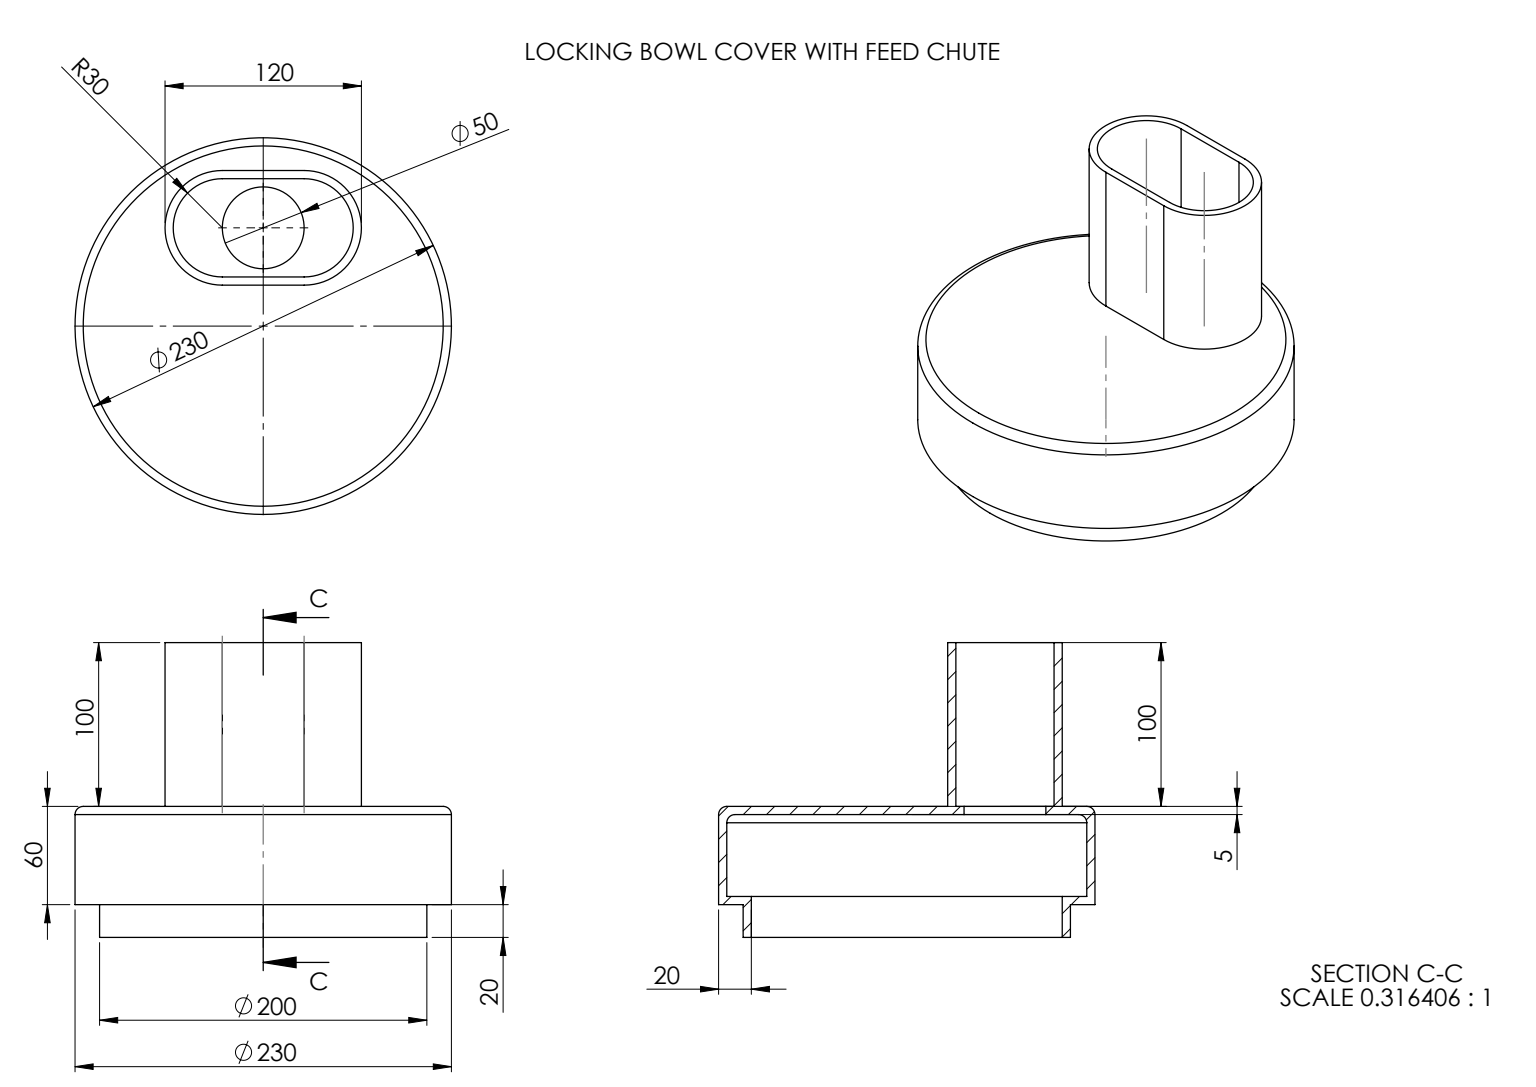
ISO-10303-21;
HEADER;
FILE_DESCRIPTION (('STEP AP214'),
    '1' );
FILE_NAME ('Locking Bowl Cover with Feed Chute.step',
    '2026-10-08T14:59:03',
    ( '' ),
    ( '' ),
    'SwSTEP 2.0',
    'SolidWorks 2026',
    '' );
FILE_SCHEMA (( 'AUTOMOTIVE_DESIGN' ));
ENDSEC;

DATA;
#12=CARTESIAN_POINT ( 'NONE',  ( -25.00000000000000000, 445.0000000000000568, -90.00000000000000000 ) ) ;
#55=DIRECTION ( 'NONE',  ( -0.000000000000000000, -1.000000000000000000, -0.000000000000000000 ) ) ;
#62=CARTESIAN_POINT ( 'NONE',  ( -25.00000000000000000, 345.0000000000000568, -90.00000000000000000 ) ) ;
#72=FACE_BOUND ( 'NONE', #11694, .T. ) ;
#91=EDGE_CURVE ( 'NONE', #9396, #343, #11975, .T. ) ;
#93=VECTOR ( 'NONE', #163, 1000.000000000000000 ) ;
#95=AXIS2_PLACEMENT_3D ( 'NONE', #7431, #12111, #3682 ) ;
#112=AXIS2_PLACEMENT_3D ( 'NONE', #12229, #2739, #12169 ) ;
#129=ORIENTED_EDGE ( 'NONE', *, *, #8171, .F. ) ;
#161=CARTESIAN_POINT ( 'NONE',  ( 0.000000000000000000, 264.9990000000000236, -34.99999999999999289 ) ) ;
#163=DIRECTION ( 'NONE',  ( -0.000000000000000000, -1.000000000000000000, -0.000000000000000000 ) ) ;
#170=ORIENTED_EDGE ( 'NONE', *, *, #8169, .T. ) ;
#173=EDGE_LOOP ( 'NONE', ( #129, #2028 ) ) ;
#209=EDGE_LOOP ( 'NONE', ( #9146, #6174, #8156, #10356 ) ) ;
#241=EDGE_LOOP ( 'NONE', ( #9519, #6626 ) ) ;
#258=ORIENTED_EDGE ( 'NONE', *, *, #4138, .F. ) ;
#290=ORIENTED_EDGE ( 'NONE', *, *, #11197, .T. ) ;
#300=DIRECTION ( 'NONE',  ( 0.000000000000000000, 1.000000000000000000, 0.000000000000000000 ) ) ;
#319=CARTESIAN_POINT ( 'NONE',  ( 25.00000000000000000, 445.0000000000000568, -59.99999999999999289 ) ) ;
#338=EDGE_CURVE ( 'NONE', #9423, #8980, #11374, .T. ) ;
#343=VERTEX_POINT ( 'NONE', #2827 ) ;
#362=ORIENTED_EDGE ( 'NONE', *, *, #8065, .F. ) ;
#365=EDGE_CURVE ( 'NONE', #6665, #9990, #8676, .T. ) ;
#366=VERTEX_POINT ( 'NONE', #3827 ) ;
#395=CARTESIAN_POINT ( 'NONE',  ( 0.000000000000000000, 290.0000000000000568, 0.000000000000000000 ) ) ;
#414=CARTESIAN_POINT ( 'NONE',  ( -25.00000000000000000, 445.0000000000000568, -24.99999999999998934 ) ) ;
#450=ORIENTED_EDGE ( 'NONE', *, *, #10797, .T. ) ;
#463=( LENGTH_UNIT ( ) NAMED_UNIT ( * ) SI_UNIT ( .MILLI., .METRE. ) );
#483=VECTOR ( 'NONE', #12060, 1000.000000000000000 ) ;
#559=EDGE_CURVE ( 'NONE', #12107, #9423, #10128, .T. ) ;
#569=FACE_OUTER_BOUND ( 'NONE', #2899, .T. ) ;
#606=AXIS2_PLACEMENT_3D ( 'NONE', #1785, #8264, #12267 ) ;
#623=CIRCLE ( 'NONE', #4397, 100.0000000000000284 ) ;
#634=CARTESIAN_POINT ( 'NONE',  ( 0.000000000000000000, 340.0000000000000000, 0.000000000000000000 ) ) ;
#645=DIRECTION ( 'NONE',  ( 0.000000000000000000, -0.000000000000000000, 1.000000000000000000 ) ) ;
#656=ORIENTED_EDGE ( 'NONE', *, *, #8171, .T. ) ;
#660=CARTESIAN_POINT ( 'NONE',  ( 0.000000000000000000, 264.9990000000000236, -59.99999999999999289 ) ) ;
#673=ORIENTED_EDGE ( 'NONE', *, *, #10831, .F. ) ;
#749=EDGE_CURVE ( 'NONE', #980, #10107, #8125, .T. ) ;
#766=LINE ( 'NONE', #6554, #1224 ) ;
#768=EDGE_LOOP ( 'NONE', ( #10087, #10275, #11943, #656 ) ) ;
#775=EDGE_CURVE ( 'NONE', #8980, #6431, #10558, .T. ) ;
#792=CARTESIAN_POINT ( 'NONE',  ( 24.99999999999999645, 445.0000000000000568, -95.00000000000000000 ) ) ;
#795=CARTESIAN_POINT ( 'NONE',  ( -25.00000000000000000, 445.0000000000000568, -90.00000000000000000 ) ) ;
#797=DIRECTION ( 'NONE',  ( -0.000000000000000000, -1.000000000000000000, -0.000000000000000000 ) ) ;
#798=ADVANCED_FACE ( 'NONE', ( #9554 ), #9306, .F. ) ;
#799=AXIS2_PLACEMENT_3D ( 'NONE', #8396, #2668, #933 ) ;
#809=CARTESIAN_POINT ( 'NONE',  ( 0.000000000000000000, 265.0000000000000000, 0.000000000000000000 ) ) ;
#826=AXIS2_PLACEMENT_3D ( 'NONE', #4284, #9299, #12253 ) ;
#839=ORIENTED_EDGE ( 'NONE', *, *, #3131, .F. ) ;
#842=VECTOR ( 'NONE', #3095, 1000.000000000000000 ) ;
#857=DIRECTION ( 'NONE',  ( 0.000000000000000000, 0.000000000000000000, -1.000000000000000000 ) ) ;
#868=VECTOR ( 'NONE', #6176, 1000.000000000000000 ) ;
#878=ORIENTED_EDGE ( 'NONE', *, *, #1877, .T. ) ;
#910=CARTESIAN_POINT ( 'NONE',  ( -25.00000000000000000, 445.0000000000000568, -90.00000000000000000 ) ) ;
#920=DIRECTION ( 'NONE',  ( -0.000000000000000000, -1.000000000000000000, -0.000000000000000000 ) ) ;
#932=DIRECTION ( 'NONE',  ( 0.000000000000000000, 0.000000000000000000, 1.000000000000000000 ) ) ;
#933=DIRECTION ( 'NONE',  ( 0.000000000000000000, 0.000000000000000000, 1.000000000000000000 ) ) ;
#962=DIRECTION ( 'NONE',  ( 0.000000000000000000, 1.000000000000000000, 0.000000000000000000 ) ) ;
#971=ORIENTED_EDGE ( 'NONE', *, *, #3981, .F. ) ;
#980=VERTEX_POINT ( 'NONE', #1154 ) ;
#994=MECHANICAL_DESIGN_GEOMETRIC_PRESENTATION_REPRESENTATION('',(#6364),#3151);
#1004=VERTEX_POINT ( 'NONE', #10865 ) ;
#1020=DIRECTION ( 'NONE',  ( -0.000000000000000000, -1.000000000000000000, -0.000000000000000000 ) ) ;
#1022=EDGE_CURVE ( 'NONE', #1669, #6843, #3206, .T. ) ;
#1047=ORIENTED_EDGE ( 'NONE', *, *, #3864, .F. ) ;
#1059=CARTESIAN_POINT ( 'NONE',  ( 0.000000000000000000, 335.0000000000000000, 0.000000000000000000 ) ) ;
#1066=CARTESIAN_POINT ( 'NONE',  ( 0.000000000000000000, 340.0000000000000000, 0.000000000000000000 ) ) ;
#1080=EDGE_CURVE ( 'NONE', #366, #8042, #4441, .T. ) ;
#1100=CIRCLE ( 'NONE', #7062, 25.00000000000000000 ) ;
#1103=ORIENTED_EDGE ( 'NONE', *, *, #4649, .T. ) ;
#1110=CARTESIAN_POINT ( 'NONE',  ( -25.00000000000000000, 445.0000000000000568, -29.99999999999999289 ) ) ;
#1114=PRODUCT_DEFINITION_SHAPE ( 'NONE', 'NONE',  #7780 ) ;
#1116=AXIS2_PLACEMENT_3D ( 'NONE', #2438, #7051, #1380 ) ;
#1128=ORIENTED_EDGE ( 'NONE', *, *, #4703, .F. ) ;
#1129=DIRECTION ( 'NONE',  ( 0.000000000000000000, 0.000000000000000000, 1.000000000000000000 ) ) ;
#1131=CARTESIAN_POINT ( 'NONE',  ( 0.000000000000000000, 340.0000000000000000, 0.000000000000000000 ) ) ;
#1154=CARTESIAN_POINT ( 'NONE',  ( 3.061616997868383043E-15, 340.0000000000000000, -84.99999999999998579 ) ) ;
#1180=DIRECTION ( 'NONE',  ( 0.000000000000000000, 0.000000000000000000, -1.000000000000000000 ) ) ;
#1192=CARTESIAN_POINT ( 'NONE',  ( 0.000000000000000000, 265.0000000000000000, 0.000000000000000000 ) ) ;
#1193=ORIENTED_EDGE ( 'NONE', *, *, #4561, .T. ) ;
#1196=ORIENTED_EDGE ( 'NONE', *, *, #3655, .T. ) ;
#1224=VECTOR ( 'NONE', #12235, 1000.000000000000000 ) ;
#1227=DIRECTION ( 'NONE',  ( 0.000000000000000000, 0.000000000000000000, 1.000000000000000000 ) ) ;
#1238=AXIS2_PLACEMENT_3D ( 'NONE', #1784, #6529, #6582 ) ;
#1248=AXIS2_PLACEMENT_3D ( 'NONE', #10310, #6332, #2532 ) ;
#1250=DIRECTION ( 'NONE',  ( 0.000000000000000000, 1.000000000000000000, 0.000000000000000000 ) ) ;
#1292=DIRECTION ( 'NONE',  ( 1.000000000000000000, 0.000000000000000000, -0.000000000000000000 ) ) ;
#1297=LINE ( 'NONE', #10769, #9355 ) ;
#1313=CLOSED_SHELL ( 'NONE', ( #3230, #7953, #9387, #12328, #9620, #5138, #7591, #4251, #2390, #5665, #9897, #798, #10427, #12260, #12222, #2538, #10180, #10873, #5121, #9944, #12231, #11960, #6025, #4909, #4674, #5505, #5178, #3185, #9915 ) ) ;
#1315=CIRCLE ( 'NONE', #5902, 35.00000000000000000 ) ;
#1317=ORIENTED_EDGE ( 'NONE', *, *, #9120, .T. ) ;
#1325=CYLINDRICAL_SURFACE ( 'NONE', #1672, 95.00000000000002842 ) ;
#1346=ORIENTED_EDGE ( 'NONE', *, *, #5064, .F. ) ;
#1380=DIRECTION ( 'NONE',  ( 0.000000000000000000, 0.000000000000000000, 1.000000000000000000 ) ) ;
#1381=ORIENTED_EDGE ( 'NONE', *, *, #10829, .T. ) ;
#1410=CARTESIAN_POINT ( 'NONE',  ( 0.000000000000000000, 340.0000000000000000, 0.000000000000000000 ) ) ;
#1422=VECTOR ( 'NONE', #9629, 1000.000000000000000 ) ;
#1427=DIRECTION ( 'NONE',  ( 0.000000000000000000, 1.000000000000000000, 0.000000000000000000 ) ) ;
#1464=PLANE ( 'NONE',  #3000 ) ;
#1475=DIRECTION ( 'NONE',  ( -0.000000000000000000, -1.000000000000000000, -0.000000000000000000 ) ) ;
#1478=DIRECTION ( 'NONE',  ( 0.000000000000000000, 0.000000000000000000, 1.000000000000000000 ) ) ;
#1485=EDGE_LOOP ( 'NONE', ( #5479, #1619 ) ) ;
#1488=CARTESIAN_POINT ( 'NONE',  ( 0.000000000000000000, 345.0000000000000568, -59.99999999999999289 ) ) ;
#1495=ORIENTED_EDGE ( 'NONE', *, *, #3254, .F. ) ;
#1496=DIRECTION ( 'NONE',  ( 0.000000000000000000, 0.000000000000000000, 1.000000000000000000 ) ) ;
#1516=EDGE_CURVE ( 'NONE', #9990, #4918, #10969, .T. ) ;
#1579=DIRECTION ( 'NONE',  ( 0.000000000000000000, 0.000000000000000000, 1.000000000000000000 ) ) ;
#1584=DIRECTION ( 'NONE',  ( 0.000000000000000000, 0.000000000000000000, 1.000000000000000000 ) ) ;
#1588=EDGE_CURVE ( 'NONE', #6133, #7105, #5611, .T. ) ;
#1591=SURFACE_STYLE_USAGE ( .BOTH. , #4385 ) ;
#1592=CIRCLE ( 'NONE', #2182, 110.0000000000000284 ) ;
#1594=FACE_OUTER_BOUND ( 'NONE', #6328, .T. ) ;
#1610=AXIS2_PLACEMENT_3D ( 'NONE', #11271, #10315, #5592 ) ;
#1612=AXIS2_PLACEMENT_3D ( 'NONE', #9562, #7823, #5032 ) ;
#1618=DIRECTION ( 'NONE',  ( 0.000000000000000000, 0.000000000000000000, 1.000000000000000000 ) ) ;
#1619=ORIENTED_EDGE ( 'NONE', *, *, #3254, .T. ) ;
#1647=ORIENTED_EDGE ( 'NONE', *, *, #9120, .F. ) ;
#1648=CARTESIAN_POINT ( 'NONE',  ( 25.00000000000000000, 345.0000000000000568, -24.99999999999998934 ) ) ;
#1668=DIRECTION ( 'NONE',  ( 0.000000000000000000, 0.000000000000000000, -1.000000000000000000 ) ) ;
#1669=VERTEX_POINT ( 'NONE', #3557 ) ;
#1672=AXIS2_PLACEMENT_3D ( 'NONE', #10853, #2316, #5437 ) ;
#1683=AXIS2_PLACEMENT_3D ( 'NONE', #10392, #1855, #932 ) ;
#1687=ORIENTED_EDGE ( 'NONE', *, *, #11584, .F. ) ;
#1702=VECTOR ( 'NONE', #8940, 1000.000000000000000 ) ;
#1713=DIRECTION ( 'NONE',  ( 0.000000000000000000, -0.000000000000000000, 1.000000000000000000 ) ) ;
#1751=EDGE_CURVE ( 'NONE', #2693, #6100, #5845, .T. ) ;
#1784=CARTESIAN_POINT ( 'NONE',  ( 0.000000000000000000, 264.9990000000000236, -59.99999999999999289 ) ) ;
#1785=CARTESIAN_POINT ( 'NONE',  ( -25.00000000000000000, 445.0000000000000568, -59.99999999999999289 ) ) ;
#1844=CARTESIAN_POINT ( 'NONE',  ( 0.000000000000000000, 340.0000000000000000, 0.000000000000000000 ) ) ;
#1850=DIRECTION ( 'NONE',  ( -1.000000000000000000, 0.000000000000000000, 0.000000000000000000 ) ) ;
#1855=DIRECTION ( 'NONE',  ( -0.000000000000000000, -1.000000000000000000, -0.000000000000000000 ) ) ;
#1859=CARTESIAN_POINT ( 'NONE',  ( -25.00000000000000000, 445.0000000000000568, -59.99999999999999289 ) ) ;
#1862=LINE ( 'NONE', #8522, #4334 ) ;
#1866=DIRECTION ( 'NONE',  ( 1.000000000000000000, 0.000000000000000000, 0.000000000000000000 ) ) ;
#1877=EDGE_CURVE ( 'NONE', #11984, #12107, #2341, .T. ) ;
#1899=PRODUCT ( 'Locking Bowl Cover with Feed Chute', 'Locking Bowl Cover with Feed Chute', '', ( #8716 ) ) ;
#1911=AXIS2_PLACEMENT_3D ( 'NONE', #10684, #11693, #3144 ) ;
#1940=DIRECTION ( 'NONE',  ( 1.000000000000000000, 0.000000000000000000, 0.000000000000000000 ) ) ;
#1958=EDGE_CURVE ( 'NONE', #12281, #3955, #5339, .T. ) ;
#1961=DIRECTION ( 'NONE',  ( -0.000000000000000000, -1.000000000000000000, -0.000000000000000000 ) ) ;
#1977=DIRECTION ( 'NONE',  ( 0.000000000000000000, 0.000000000000000000, 1.000000000000000000 ) ) ;
#1986=CARTESIAN_POINT ( 'NONE',  ( -25.00000000000000000, 445.0000000000000568, -29.99999999999999289 ) ) ;
#2004=AXIS2_PLACEMENT_3D ( 'NONE', #8641, #10522, #1180 ) ;
#2024=TOROIDAL_SURFACE ( 'NONE', #8969, 110.0000000000000284, 5.000000000000000000 ) ;
#2028=ORIENTED_EDGE ( 'NONE', *, *, #7862, .F. ) ;
#2060=DIRECTION ( 'NONE',  ( 0.000000000000000000, 1.000000000000000000, 0.000000000000000000 ) ) ;
#2064=VERTEX_POINT ( 'NONE', #9558 ) ;
#2098=AXIS2_PLACEMENT_3D ( 'NONE', #2517, #5324, #1579 ) ;
#2117=FACE_OUTER_BOUND ( 'NONE', #209, .T. ) ;
#2138=CARTESIAN_POINT ( 'NONE',  ( 1.408343819019456413E-14, 285.0000000000000568, 115.0000000000000284 ) ) ;
#2142=LINE ( 'NONE', #2197, #2388 ) ;
#2182=AXIS2_PLACEMENT_3D ( 'NONE', #2553, #6356, #1496 ) ;
#2197=CARTESIAN_POINT ( 'NONE',  ( -25.00000000000000000, 445.0000000000000568, -24.99999999999998934 ) ) ;
#2213=AXIS2_PLACEMENT_3D ( 'NONE', #1131, #55, #10532 ) ;
#2262=AXIS2_PLACEMENT_3D ( 'NONE', #3647, #12199, #5711 ) ;
#2263=AXIS2_PLACEMENT_3D ( 'NONE', #6307, #4185, #3445 ) ;
#2269=DIRECTION ( 'NONE',  ( 0.000000000000000000, 0.000000000000000000, 1.000000000000000000 ) ) ;
#2285=( LENGTH_UNIT ( ) NAMED_UNIT ( * ) SI_UNIT ( .MILLI., .METRE. ) );
#2301=CARTESIAN_POINT ( 'NONE',  ( -25.00000000000000000, 445.0000000000000568, -59.99999999999999289 ) ) ;
#2316=DIRECTION ( 'NONE',  ( 0.000000000000000000, 1.000000000000000000, 0.000000000000000000 ) ) ;
#2341=LINE ( 'NONE', #4034, #842 ) ;
#2342=PRESENTATION_STYLE_ASSIGNMENT (( #11772 ) ) ;
#2355=DIRECTION ( 'NONE',  ( 0.000000000000000000, 1.000000000000000000, 0.000000000000000000 ) ) ;
#2365=ORIENTED_EDGE ( 'NONE', *, *, #1877, .F. ) ;
#2388=VECTOR ( 'NONE', #5945, 1000.000000000000000 ) ;
#2389=FACE_OUTER_BOUND ( 'NONE', #3479, .T. ) ;
#2390=ADVANCED_FACE ( 'NONE', ( #10930, #2389 ), #1464, .T. ) ;
#2394=ORIENTED_EDGE ( 'NONE', *, *, #8117, .F. ) ;
#2438=CARTESIAN_POINT ( 'NONE',  ( 0.000000000000000000, 335.0000000000000000, 105.0000000000000284 ) ) ;
#2462=( NAMED_UNIT ( * ) PLANE_ANGLE_UNIT ( ) SI_UNIT ( $, .RADIAN. ) );
#2476=DIRECTION ( 'NONE',  ( 1.000000000000000000, 0.000000000000000000, 0.000000000000000000 ) ) ;
#2484=ORIENTED_EDGE ( 'NONE', *, *, #1751, .T. ) ;
#2514=CIRCLE ( 'NONE', #6297, 95.00000000000002842 ) ;
#2516=FACE_BOUND ( 'NONE', #241, .T. ) ;
#2517=CARTESIAN_POINT ( 'NONE',  ( 0.000000000000000000, 340.0000000000000000, -59.99999999999999289 ) ) ;
#2532=DIRECTION ( 'NONE',  ( 0.000000000000000000, 0.000000000000000000, 1.000000000000000000 ) ) ;
#2538=ADVANCED_FACE ( 'NONE', ( #2516, #12121 ), #5633, .F. ) ;
#2553=CARTESIAN_POINT ( 'NONE',  ( 0.000000000000000000, 335.0000000000000000, 0.000000000000000000 ) ) ;
#2595=EDGE_CURVE ( 'NONE', #10953, #6431, #2877, .T. ) ;
#2601=DIRECTION ( 'NONE',  ( -0.000000000000000000, -1.000000000000000000, -0.000000000000000000 ) ) ;
#2607=VERTEX_POINT ( 'NONE', #11365 ) ;
#2635=EDGE_LOOP ( 'NONE', ( #7285, #5878, #878, #11411 ) ) ;
#2643=EDGE_LOOP ( 'NONE', ( #5773, #6443, #6520, #10027 ) ) ;
#2668=DIRECTION ( 'NONE',  ( -0.000000000000000000, -1.000000000000000000, -0.000000000000000000 ) ) ;
#2681=AXIS2_PLACEMENT_3D ( 'NONE', #11662, #3113, #7033 ) ;
#2693=VERTEX_POINT ( 'NONE', #11425 ) ;
#2696=ORIENTED_EDGE ( 'NONE', *, *, #7107, .F. ) ;
#2718=CYLINDRICAL_SURFACE ( 'NONE', #8556, 110.0000000000000284 ) ;
#2739=DIRECTION ( 'NONE',  ( 0.000000000000000000, 1.000000000000000000, 0.000000000000000000 ) ) ;
#2770=CIRCLE ( 'NONE', #10938, 30.00000000000000355 ) ;
#2774=DIRECTION ( 'NONE',  ( 0.000000000000000000, 1.000000000000000000, 0.000000000000000000 ) ) ;
#2779=UNCERTAINTY_MEASURE_WITH_UNIT (LENGTH_MEASURE( 1.000000000000000082E-05 ), #12007, 'distance_accuracy_value', 'NONE');
#2804=EDGE_LOOP ( 'NONE', ( #12277, #1128, #3707, #3241 ) ) ;
#2826=FACE_BOUND ( 'NONE', #7544, .T. ) ;
#2827=CARTESIAN_POINT ( 'NONE',  ( -25.00000000000000000, 445.0000000000000568, -24.99999999999998934 ) ) ;
#2858=VECTOR ( 'NONE', #10914, 1000.000000000000000 ) ;
#2869=DIRECTION ( 'NONE',  ( 0.000000000000000000, 1.000000000000000000, 0.000000000000000000 ) ) ;
#2877=LINE ( 'NONE', #62, #5369 ) ;
#2899=EDGE_LOOP ( 'NONE', ( #8408, #5265, #5179, #1687 ) ) ;
#2901=MECHANICAL_DESIGN_GEOMETRIC_PRESENTATION_REPRESENTATION('',(#10655),#9649);
#2904=FACE_OUTER_BOUND ( 'NONE', #5361, .T. ) ;
#2916=DIRECTION ( 'NONE',  ( 0.000000000000000000, 1.000000000000000000, 0.000000000000000000 ) ) ;
#2951=PLANE ( 'NONE',  #5593 ) ;
#2959=ORIENTED_EDGE ( 'NONE', *, *, #365, .F. ) ;
#2985=CYLINDRICAL_SURFACE ( 'NONE', #2004, 35.00000000000000711 ) ;
#2991=DIRECTION ( 'NONE',  ( 0.000000000000000000, 1.000000000000000000, 0.000000000000000000 ) ) ;
#3000=AXIS2_PLACEMENT_3D ( 'NONE', #5270, #9049, #8056 ) ;
#3001=EDGE_CURVE ( 'NONE', #11680, #10543, #9583, .T. ) ;
#3004=EDGE_CURVE ( 'NONE', #8712, #8042, #1862, .T. ) ;
#3022=CARTESIAN_POINT ( 'NONE',  ( 25.00000000000000000, 445.0000000000000568, -59.99999999999999289 ) ) ;
#3047=ORIENTED_EDGE ( 'NONE', *, *, #8065, .T. ) ;
#3069=EDGE_LOOP ( 'NONE', ( #8765, #5742, #9232, #10691 ) ) ;
#3080=EDGE_LOOP ( 'NONE', ( #9286, #4717, #12223, #3130 ) ) ;
#3095=DIRECTION ( 'NONE',  ( 1.000000000000000000, 0.000000000000000000, 0.000000000000000000 ) ) ;
#3097=( NAMED_UNIT ( * ) PLANE_ANGLE_UNIT ( ) SI_UNIT ( $, .RADIAN. ) );
#3104=CIRCLE ( 'NONE', #4504, 35.00000000000000000 ) ;
#3113=DIRECTION ( 'NONE',  ( 1.000000000000000000, -0.000000000000000000, 1.224646799147353207E-16 ) ) ;
#3118=DIRECTION ( 'NONE',  ( 0.000000000000000000, 0.000000000000000000, 1.000000000000000000 ) ) ;
#3130=ORIENTED_EDGE ( 'NONE', *, *, #775, .T. ) ;
#3131=EDGE_CURVE ( 'NONE', #7450, #7160, #6738, .T. ) ;
#3136=ORIENTED_EDGE ( 'NONE', *, *, #9839, .F. ) ;
#3144=DIRECTION ( 'NONE',  ( 0.000000000000000000, 0.000000000000000000, 1.000000000000000000 ) ) ;
#3151=( GEOMETRIC_REPRESENTATION_CONTEXT ( 3 ) GLOBAL_UNCERTAINTY_ASSIGNED_CONTEXT ( ( #2779 ) ) GLOBAL_UNIT_ASSIGNED_CONTEXT ( ( #12007, #5397, #3462 ) ) REPRESENTATION_CONTEXT ( 'NONE', 'WORKASPACE' ) );
#3170=CARTESIAN_POINT ( 'NONE',  ( 0.000000000000000000, 345.0000000000000568, 0.000000000000000000 ) ) ;
#3176=( GEOMETRIC_REPRESENTATION_CONTEXT ( 3 ) GLOBAL_UNCERTAINTY_ASSIGNED_CONTEXT ( ( #10383 ) ) GLOBAL_UNIT_ASSIGNED_CONTEXT ( ( #463, #2462, #11701 ) ) REPRESENTATION_CONTEXT ( 'NONE', 'WORKASPACE' ) );
#3185=ADVANCED_FACE ( 'NONE', ( #1594 ), #6914, .F. ) ;
#3206=LINE ( 'NONE', #7008, #9424 ) ;
#3230=ADVANCED_FACE ( 'NONE', ( #2117 ), #6212, .F. ) ;
#3241=ORIENTED_EDGE ( 'NONE', *, *, #1958, .T. ) ;
#3254=EDGE_CURVE ( 'NONE', #7160, #2064, #7135, .T. ) ;
#3286=DIRECTION ( 'NONE',  ( -1.000000000000000000, 0.000000000000000000, -0.000000000000000000 ) ) ;
#3313=CARTESIAN_POINT ( 'NONE',  ( 0.000000000000000000, 285.0000000000000568, 0.000000000000000000 ) ) ;
#3332=DIRECTION ( 'NONE',  ( 0.000000000000000000, 1.000000000000000000, 0.000000000000000000 ) ) ;
#3381=EDGE_LOOP ( 'NONE', ( #12170, #10802, #290, #3617 ) ) ;
#3395=CARTESIAN_POINT ( 'NONE',  ( 0.000000000000000000, 335.0000000000000000, 0.000000000000000000 ) ) ;
#3396=AXIS2_PLACEMENT_3D ( 'NONE', #6373, #4310, #4434 ) ;
#3407=DIRECTION ( 'NONE',  ( 0.000000000000000000, 0.000000000000000000, 1.000000000000000000 ) ) ;
#3419=AXIS2_PLACEMENT_3D ( 'NONE', #5370, #10033, #9088 ) ;
#3429=FACE_OUTER_BOUND ( 'NONE', #11155, .T. ) ;
#3442=DIRECTION ( 'NONE',  ( 0.000000000000000000, 1.000000000000000000, 0.000000000000000000 ) ) ;
#3445=DIRECTION ( 'NONE',  ( 0.000000000000000000, 0.000000000000000000, 1.000000000000000000 ) ) ;
#3451=DIRECTION ( 'NONE',  ( 0.000000000000000000, 1.000000000000000000, 0.000000000000000000 ) ) ;
#3462=( NAMED_UNIT ( * ) SI_UNIT ( $, .STERADIAN. ) SOLID_ANGLE_UNIT ( ) );
#3465=VECTOR ( 'NONE', #1961, 1000.000000000000000 ) ;
#3468=CYLINDRICAL_SURFACE ( 'NONE', #1248, 100.0000000000000284 ) ;
#3476=CARTESIAN_POINT ( 'NONE',  ( 0.000000000000000000, 340.0000000000000000, 0.000000000000000000 ) ) ;
#3479=EDGE_LOOP ( 'NONE', ( #8081, #6491 ) ) ;
#3491=AXIS2_PLACEMENT_3D ( 'NONE', #7846, #2060, #1129 ) ;
#3497=DIRECTION ( 'NONE',  ( 0.000000000000000000, 0.000000000000000000, 1.000000000000000000 ) ) ;
#3528=AXIS2_PLACEMENT_3D ( 'NONE', #634, #5563, #9217 ) ;
#3540=EDGE_CURVE ( 'NONE', #4918, #9990, #9256, .T. ) ;
#3541=EDGE_CURVE ( 'NONE', #366, #12281, #3104, .T. ) ;
#3555=ORIENTED_EDGE ( 'NONE', *, *, #3004, .T. ) ;
#3557=CARTESIAN_POINT ( 'NONE',  ( 1.347111479062088996E-14, 335.0000000000000000, 110.0000000000000284 ) ) ;
#3563=CARTESIAN_POINT ( 'NONE',  ( 0.000000000000000000, 265.0000000000000000, 95.00000000000002842 ) ) ;
#3617=ORIENTED_EDGE ( 'NONE', *, *, #2595, .T. ) ;
#3633=ORIENTED_EDGE ( 'NONE', *, *, #559, .F. ) ;
#3647=CARTESIAN_POINT ( 'NONE',  ( 0.000000000000000000, 265.0000000000000000, 0.000000000000000000 ) ) ;
#3655=EDGE_CURVE ( 'NONE', #2607, #4918, #12061, .T. ) ;
#3657=CARTESIAN_POINT ( 'NONE',  ( 24.99999999999999645, 445.0000000000000568, -95.00000000000000000 ) ) ;
#3673=CIRCLE ( 'NONE', #1683, 25.00000000000000000 ) ;
#3681=AXIS2_PLACEMENT_3D ( 'NONE', #3170, #2355, #6161 ) ;
#3682=DIRECTION ( 'NONE',  ( 1.000000000000000000, 0.000000000000000000, 0.000000000000000000 ) ) ;
#3684=ORIENTED_EDGE ( 'NONE', *, *, #10831, .T. ) ;
#3697=VECTOR ( 'NONE', #7382, 1000.000000000000000 ) ;
#3707=ORIENTED_EDGE ( 'NONE', *, *, #8169, .F. ) ;
#3715=PLANE ( 'NONE',  #606 ) ;
#3734=DIRECTION ( 'NONE',  ( -0.000000000000000000, -1.000000000000000000, -0.000000000000000000 ) ) ;
#3758=DIRECTION ( 'NONE',  ( 0.000000000000000000, 0.000000000000000000, 1.000000000000000000 ) ) ;
#3764=ORIENTED_EDGE ( 'NONE', *, *, #3131, .T. ) ;
#3787=ORIENTED_EDGE ( 'NONE', *, *, #91, .T. ) ;
#3827=CARTESIAN_POINT ( 'NONE',  ( 25.00000000000000000, 445.0000000000000568, -24.99999999999998934 ) ) ;
#3843=VECTOR ( 'NONE', #3734, 1000.000000000000000 ) ;
#3845=CARTESIAN_POINT ( 'NONE',  ( 0.000000000000000000, 265.0000000000000000, 100.0000000000000284 ) ) ;
#3858=CIRCLE ( 'NONE', #3491, 100.0000000000000284 ) ;
#3864=EDGE_CURVE ( 'NONE', #1669, #2064, #6492, .T. ) ;
#3866=DIRECTION ( 'NONE',  ( 0.000000000000000000, 0.000000000000000000, 1.000000000000000000 ) ) ;
#3874=AXIS2_PLACEMENT_3D ( 'NONE', #809, #7416, #11218 ) ;
#3898=EDGE_LOOP ( 'NONE', ( #3787, #7824, #11739, #170 ) ) ;
#3906=DIRECTION ( 'NONE',  ( -0.000000000000000000, 0.000000000000000000, 1.000000000000000000 ) ) ;
#3933=DIRECTION ( 'NONE',  ( 0.000000000000000000, 1.000000000000000000, 0.000000000000000000 ) ) ;
#3955=VERTEX_POINT ( 'NONE', #8098 ) ;
#3981=EDGE_CURVE ( 'NONE', #10107, #6100, #7093, .T. ) ;
#3994=DIRECTION ( 'NONE',  ( 0.000000000000000000, 0.000000000000000000, 1.000000000000000000 ) ) ;
#4030=AXIS2_PLACEMENT_3D ( 'NONE', #3395, #5679, #1584 ) ;
#4034=CARTESIAN_POINT ( 'NONE',  ( -25.00000000000000000, 445.0000000000000568, -29.99999999999999289 ) ) ;
#4037=LINE ( 'NONE', #11897, #1702 ) ;
#4052=CARTESIAN_POINT ( 'NONE',  ( 25.00000000000000000, 345.0000000000000568, -29.99999999999998934 ) ) ;
#4095=PLANE ( 'NONE',  #12067 ) ;
#4112=DIRECTION ( 'NONE',  ( 0.000000000000000000, 0.000000000000000000, -1.000000000000000000 ) ) ;
#4114=LINE ( 'NONE', #8594, #10164 ) ;
#4115=EDGE_CURVE ( 'NONE', #6843, #1004, #6870, .T. ) ;
#4129=DIRECTION ( 'NONE',  ( 0.000000000000000000, 1.000000000000000000, 0.000000000000000000 ) ) ;
#4138=EDGE_CURVE ( 'NONE', #7105, #11220, #11538, .T. ) ;
#4146=AXIS2_PLACEMENT_3D ( 'NONE', #7722, #11535, #6605 ) ;
#4185=DIRECTION ( 'NONE',  ( 0.000000000000000000, 1.000000000000000000, 0.000000000000000000 ) ) ;
#4213=EDGE_CURVE ( 'NONE', #6665, #7233, #5280, .T. ) ;
#4251=ADVANCED_FACE ( 'NONE', ( #8021, #10897 ), #5984, .T. ) ;
#4266=EDGE_CURVE ( 'NONE', #6100, #10107, #1100, .T. ) ;
#4284=CARTESIAN_POINT ( 'NONE',  ( -25.00000000000000000, 445.0000000000000568, -59.99999999999999289 ) ) ;
#4302=VERTEX_POINT ( 'NONE', #4052 ) ;
#4309=ORIENTED_EDGE ( 'NONE', *, *, #6724, .T. ) ;
#4310=DIRECTION ( 'NONE',  ( -1.000000000000000000, 0.000000000000000000, 0.000000000000000000 ) ) ;
#4334=VECTOR ( 'NONE', #4925, 1000.000000000000000 ) ;
#4336=FACE_OUTER_BOUND ( 'NONE', #10270, .T. ) ;
#4371=CIRCLE ( 'NONE', #3396, 5.000000000000004441 ) ;
#4385=SURFACE_SIDE_STYLE ('',( #11069 ) ) ;
#4393=CARTESIAN_POINT ( 'NONE',  ( 25.00000000000000000, 445.0000000000000568, -59.99999999999999289 ) ) ;
#4397=AXIS2_PLACEMENT_3D ( 'NONE', #1192, #1250, #3994 ) ;
#4400=LINE ( 'NONE', #8195, #7063 ) ;
#4409=VERTEX_POINT ( 'NONE', #10200 ) ;
#4430=DIRECTION ( 'NONE',  ( -1.000000000000000000, 0.000000000000000000, -0.000000000000000000 ) ) ;
#4434=DIRECTION ( 'NONE',  ( 0.000000000000000000, 0.000000000000000000, 1.000000000000000000 ) ) ;
#4441=LINE ( 'NONE', #11937, #483 ) ;
#4451=EDGE_LOOP ( 'NONE', ( #8123, #673, #10360, #1647 ) ) ;
#4484=EDGE_LOOP ( 'NONE', ( #2365, #11020, #10902, #3633 ) ) ;
#4487=CARTESIAN_POINT ( 'NONE',  ( 25.00000000000000000, 445.0000000000000568, -90.00000000000000000 ) ) ;
#4497=FACE_OUTER_BOUND ( 'NONE', #2635, .T. ) ;
#4498=VECTOR ( 'NONE', #10653, 1000.000000000000000 ) ;
#4504=AXIS2_PLACEMENT_3D ( 'NONE', #3022, #11568, #7756 ) ;
#4557=ORIENTED_EDGE ( 'NONE', *, *, #11197, .F. ) ;
#4561=EDGE_CURVE ( 'NONE', #11110, #7233, #11457, .T. ) ;
#4586=FACE_BOUND ( 'NONE', #7622, .T. ) ;
#4590=CARTESIAN_POINT ( 'NONE',  ( 0.000000000000000000, 290.0000000000000568, 0.000000000000000000 ) ) ;
#4634=CIRCLE ( 'NONE', #11614, 95.00000000000002842 ) ;
#4649=EDGE_CURVE ( 'NONE', #11984, #11751, #9631, .T. ) ;
#4650=VERTEX_POINT ( 'NONE', #11588 ) ;
#4674=ADVANCED_FACE ( 'NONE', ( #5161 ), #4095, .F. ) ;
#4689=ORIENTED_EDGE ( 'NONE', *, *, #8117, .T. ) ;
#4703=EDGE_CURVE ( 'NONE', #9396, #4409, #4037, .T. ) ;
#4709=MANIFOLD_SOLID_BREP ( 'Extrude-Thin3', #1313 ) ;
#4711=FACE_OUTER_BOUND ( 'NONE', #8267, .T. ) ;
#4717=ORIENTED_EDGE ( 'NONE', *, *, #6724, .F. ) ;
#4730=ORIENTED_EDGE ( 'NONE', *, *, #10868, .F. ) ;
#4731=CARTESIAN_POINT ( 'NONE',  ( 0.000000000000000000, 290.0000000000000568, 0.000000000000000000 ) ) ;
#4824=CARTESIAN_POINT ( 'NONE',  ( 0.000000000000000000, 290.0000000000000568, -115.0000000000000284 ) ) ;
#4828=VERTEX_POINT ( 'NONE', #8316 ) ;
#4850=ORIENTED_EDGE ( 'NONE', *, *, #5364, .F. ) ;
#4863=DIRECTION ( 'NONE',  ( 1.000000000000000000, 0.000000000000000000, 0.000000000000000000 ) ) ;
#4878=DIRECTION ( 'NONE',  ( -1.000000000000000000, 0.000000000000000000, -0.000000000000000000 ) ) ;
#4909=ADVANCED_FACE ( 'NONE', ( #9666 ), #8850, .T. ) ;
#4918=VERTEX_POINT ( 'NONE', #2138 ) ;
#4925=DIRECTION ( 'NONE',  ( 1.000000000000000000, 0.000000000000000000, 0.000000000000000000 ) ) ;
#4928=DIRECTION ( 'NONE',  ( 0.000000000000000000, 1.000000000000000000, 0.000000000000000000 ) ) ;
#4929=DIRECTION ( 'NONE',  ( 0.000000000000000000, 1.000000000000000000, 0.000000000000000000 ) ) ;
#4954=AXIS2_PLACEMENT_3D ( 'NONE', #660, #8772, #5337 ) ;
#4968=ORIENTED_EDGE ( 'NONE', *, *, #12131, .F. ) ;
#4984=DIRECTION ( 'NONE',  ( -0.000000000000000000, -1.000000000000000000, -0.000000000000000000 ) ) ;
#5026=AXIS2_PLACEMENT_3D ( 'NONE', #11390, #2774, #12205 ) ;
#5032=DIRECTION ( 'NONE',  ( 1.000000000000000000, 0.000000000000000000, 0.000000000000000000 ) ) ;
#5064=EDGE_CURVE ( 'NONE', #12107, #4302, #7918, .T. ) ;
#5091=CARTESIAN_POINT ( 'NONE',  ( 3.061616997868383043E-15, 345.0000000000000568, -84.99999999999998579 ) ) ;
#5103=SURFACE_STYLE_FILL_AREA ( #7945 ) ;
#5109=DIRECTION ( 'NONE',  ( 0.000000000000000000, 1.000000000000000000, 0.000000000000000000 ) ) ;
#5121=ADVANCED_FACE ( 'NONE', ( #5134 ), #11862, .F. ) ;
#5134=FACE_OUTER_BOUND ( 'NONE', #8048, .T. ) ;
#5138=ADVANCED_FACE ( 'NONE', ( #6061 ), #1325, .F. ) ;
#5157=EDGE_LOOP ( 'NONE', ( #10734, #4850, #2696, #362 ) ) ;
#5161=FACE_OUTER_BOUND ( 'NONE', #2804, .T. ) ;
#5169=ORIENTED_EDGE ( 'NONE', *, *, #6540, .F. ) ;
#5178=ADVANCED_FACE ( 'NONE', ( #4497 ), #11357, .T. ) ;
#5179=ORIENTED_EDGE ( 'NONE', *, *, #4561, .F. ) ;
#5181=EDGE_CURVE ( 'NONE', #9447, #11680, #5490, .T. ) ;
#5255=ORIENTED_EDGE ( 'NONE', *, *, #11486, .F. ) ;
#5264=AXIS2_PLACEMENT_3D ( 'NONE', #2301, #8148, #4112 ) ;
#5265=ORIENTED_EDGE ( 'NONE', *, *, #4213, .T. ) ;
#5270=CARTESIAN_POINT ( 'NONE',  ( 0.000000000000000000, 290.0000000000000568, 0.000000000000000000 ) ) ;
#5280=CIRCLE ( 'NONE', #2681, 5.000000000000004441 ) ;
#5315=CARTESIAN_POINT ( 'NONE',  ( 0.000000000000000000, 340.0000000000000000, 0.000000000000000000 ) ) ;
#5324=DIRECTION ( 'NONE',  ( -0.000000000000000000, -1.000000000000000000, -0.000000000000000000 ) ) ;
#5337=DIRECTION ( 'NONE',  ( 0.000000000000000000, 0.000000000000000000, 1.000000000000000000 ) ) ;
#5339=LINE ( 'NONE', #792, #6805 ) ;
#5361=EDGE_LOOP ( 'NONE', ( #10017, #11912, #2484, #7441 ) ) ;
#5364=EDGE_CURVE ( 'NONE', #4409, #8712, #5684, .T. ) ;
#5369=VECTOR ( 'NONE', #4878, 1000.000000000000000 ) ;
#5370=CARTESIAN_POINT ( 'NONE',  ( 0.000000000000000000, 265.0000000000000000, 0.000000000000000000 ) ) ;
#5379=AXIS2_PLACEMENT_3D ( 'NONE', #1859, #12282, #5672 ) ;
#5397=( NAMED_UNIT ( * ) PLANE_ANGLE_UNIT ( ) SI_UNIT ( $, .RADIAN. ) );
#5402=EDGE_CURVE ( 'NONE', #4828, #11220, #3858, .T. ) ;
#5437=DIRECTION ( 'NONE',  ( 0.000000000000000000, 0.000000000000000000, 1.000000000000000000 ) ) ;
#5455=CARTESIAN_POINT ( 'NONE',  ( 25.00000000000000000, 345.0000000000000568, -59.99999999999999289 ) ) ;
#5479=ORIENTED_EDGE ( 'NONE', *, *, #10585, .T. ) ;
#5490=CIRCLE ( 'NONE', #95, 95.00000000000002842 ) ;
#5505=ADVANCED_FACE ( 'NONE', ( #3429 ), #9774, .F. ) ;
#5534=PLANE ( 'NONE',  #5026 ) ;
#5542=CARTESIAN_POINT ( 'NONE',  ( -25.00000000000000000, 345.0000000000000568, -95.00000000000000000 ) ) ;
#5563=DIRECTION ( 'NONE',  ( 0.000000000000000000, 1.000000000000000000, 0.000000000000000000 ) ) ;
#5592=DIRECTION ( 'NONE',  ( 1.000000000000000000, 0.000000000000000000, 0.000000000000000000 ) ) ;
#5593=AXIS2_PLACEMENT_3D ( 'NONE', #5943, #4129, #5824 ) ;
#5611=CIRCLE ( 'NONE', #3419, 100.0000000000000284 ) ;
#5633=PLANE ( 'NONE',  #5963 ) ;
#5665=ADVANCED_FACE ( 'NONE', ( #9324 ), #10204, .T. ) ;
#5670=CARTESIAN_POINT ( 'NONE',  ( 25.00000000000000000, 345.0000000000000568, -59.99999999999999289 ) ) ;
#5672=DIRECTION ( 'NONE',  ( 0.000000000000000000, 0.000000000000000000, 1.000000000000000000 ) ) ;
#5676=LINE ( 'NONE', #4487, #3843 ) ;
#5679=DIRECTION ( 'NONE',  ( 0.000000000000000000, 1.000000000000000000, 0.000000000000000000 ) ) ;
#5682=AXIS2_PLACEMENT_3D ( 'NONE', #4731, #4928, #4863 ) ;
#5684=CIRCLE ( 'NONE', #11432, 35.00000000000000000 ) ;
#5711=DIRECTION ( 'NONE',  ( 0.000000000000000000, 0.000000000000000000, 1.000000000000000000 ) ) ;
#5721=CIRCLE ( 'NONE', #7103, 110.0000000000000284 ) ;
#5742=ORIENTED_EDGE ( 'NONE', *, *, #4138, .T. ) ;
#5773=ORIENTED_EDGE ( 'NONE', *, *, #1022, .F. ) ;
#5794=FACE_OUTER_BOUND ( 'NONE', #9070, .T. ) ;
#5805=AXIS2_PLACEMENT_3D ( 'NONE', #5315, #6124, #11868 ) ;
#5824=DIRECTION ( 'NONE',  ( 0.000000000000000000, -0.000000000000000000, 1.000000000000000000 ) ) ;
#5845=LINE ( 'NONE', #161, #1422 ) ;
#5878=ORIENTED_EDGE ( 'NONE', *, *, #4649, .F. ) ;
#5902=AXIS2_PLACEMENT_3D ( 'NONE', #5455, #8305, #1866 ) ;
#5905=EDGE_CURVE ( 'NONE', #980, #2693, #3673, .T. ) ;
#5927=DIRECTION ( 'NONE',  ( 0.000000000000000000, 1.000000000000000000, 0.000000000000000000 ) ) ;
#5943=CARTESIAN_POINT ( 'NONE',  ( 0.000000000000000000, 285.0000000000000568, 0.000000000000000000 ) ) ;
#5945=DIRECTION ( 'NONE',  ( 1.000000000000000000, 0.000000000000000000, 0.000000000000000000 ) ) ;
#5963=AXIS2_PLACEMENT_3D ( 'NONE', #8478, #3451, #645 ) ;
#5967=CARTESIAN_POINT ( 'NONE',  ( -25.00000000000000000, 445.0000000000000568, -95.00000000000000000 ) ) ;
#5981=AXIS2_PLACEMENT_3D ( 'NONE', #1844, #797, #11140 ) ;
#5984=PLANE ( 'NONE',  #3681 ) ;
#6004=FACE_OUTER_BOUND ( 'NONE', #6813, .T. ) ;
#6014=PRODUCT_DEFINITION_CONTEXT ( 'detailed design', #9946, 'design' ) ;
#6025=ADVANCED_FACE ( 'NONE', ( #4336 ), #10946, .F. ) ;
#6054=EDGE_CURVE ( 'NONE', #11751, #4302, #4400, .T. ) ;
#6061=FACE_OUTER_BOUND ( 'NONE', #8480, .T. ) ;
#6070=CARTESIAN_POINT ( 'NONE',  ( 0.000000000000000000, 345.0000000000000568, -34.99999999999999289 ) ) ;
#6100=VERTEX_POINT ( 'NONE', #6070 ) ;
#6115=ORIENTED_EDGE ( 'NONE', *, *, #5364, .T. ) ;
#6124=DIRECTION ( 'NONE',  ( -0.000000000000000000, -1.000000000000000000, -0.000000000000000000 ) ) ;
#6133=VERTEX_POINT ( 'NONE', #3845 ) ;
#6161=DIRECTION ( 'NONE',  ( 0.000000000000000000, -0.000000000000000000, 1.000000000000000000 ) ) ;
#6174=ORIENTED_EDGE ( 'NONE', *, *, #749, .T. ) ;
#6176=DIRECTION ( 'NONE',  ( -0.000000000000000000, -1.000000000000000000, -0.000000000000000000 ) ) ;
#6212=CYLINDRICAL_SURFACE ( 'NONE', #4954, 25.00000000000000000 ) ;
#6217=DIRECTION ( 'NONE',  ( 0.000000000000000000, 1.000000000000000000, 0.000000000000000000 ) ) ;
#6225=ORIENTED_EDGE ( 'NONE', *, *, #1022, .T. ) ;
#6250=EDGE_LOOP ( 'NONE', ( #3047, #9900, #12026, #6867 ) ) ;
#6256=EDGE_CURVE ( 'NONE', #2693, #980, #12257, .T. ) ;
#6297=AXIS2_PLACEMENT_3D ( 'NONE', #6918, #300, #3866 ) ;
#6307=CARTESIAN_POINT ( 'NONE',  ( 0.000000000000000000, 335.0000000000000000, 0.000000000000000000 ) ) ;
#6320=ORIENTED_EDGE ( 'NONE', *, *, #11812, .T. ) ;
#6328=EDGE_LOOP ( 'NONE', ( #4557, #1346, #6822, #4309 ) ) ;
#6332=DIRECTION ( 'NONE',  ( 0.000000000000000000, 1.000000000000000000, 0.000000000000000000 ) ) ;
#6342=DIRECTION ( 'NONE',  ( 0.000000000000000000, 0.000000000000000000, -1.000000000000000000 ) ) ;
#6356=DIRECTION ( 'NONE',  ( 0.000000000000000000, 1.000000000000000000, 0.000000000000000000 ) ) ;
#6357=EDGE_LOOP ( 'NONE', ( #11590, #11028 ) ) ;
#6364=STYLED_ITEM ( 'NONE', ( #6521 ), #11228 ) ;
#6373=CARTESIAN_POINT ( 'NONE',  ( 0.000000000000000000, 340.0000000000000000, 110.0000000000000284 ) ) ;
#6402=CARTESIAN_POINT ( 'NONE',  ( -25.00000000000000000, 345.0000000000000568, -59.99999999999999289 ) ) ;
#6431=VERTEX_POINT ( 'NONE', #8844 ) ;
#6443=ORIENTED_EDGE ( 'NONE', *, *, #11700, .T. ) ;
#6452=FILL_AREA_STYLE ('',( #8311 ) ) ;
#6469=VECTOR ( 'NONE', #2991, 1000.000000000000000 ) ;
#6491=ORIENTED_EDGE ( 'NONE', *, *, #4115, .T. ) ;
#6492=CIRCLE ( 'NONE', #1116, 5.000000000000004441 ) ;
#6520=ORIENTED_EDGE ( 'NONE', *, *, #6540, .T. ) ;
#6521=PRESENTATION_STYLE_ASSIGNMENT (( #1591 ) ) ;
#6524=ORIENTED_EDGE ( 'NONE', *, *, #11109, .T. ) ;
#6529=DIRECTION ( 'NONE',  ( -0.000000000000000000, 1.000000000000000000, -0.000000000000000000 ) ) ;
#6530=CYLINDRICAL_SURFACE ( 'NONE', #5981, 110.0000000000000284 ) ;
#6540=EDGE_CURVE ( 'NONE', #7450, #1004, #8217, .T. ) ;
#6554=CARTESIAN_POINT ( 'NONE',  ( -25.00000000000000000, 445.0000000000000568, -24.99999999999998934 ) ) ;
#6567=FACE_OUTER_BOUND ( 'NONE', #3381, .T. ) ;
#6582=DIRECTION ( 'NONE',  ( 0.000000000000000000, 0.000000000000000000, 1.000000000000000000 ) ) ;
#6586=FACE_OUTER_BOUND ( 'NONE', #6976, .T. ) ;
#6605=DIRECTION ( 'NONE',  ( 1.224646799147352468E-16, 0.000000000000000000, -1.000000000000000000 ) ) ;
#6610=ORIENTED_EDGE ( 'NONE', *, *, #4703, .T. ) ;
#6623=ORIENTED_EDGE ( 'NONE', *, *, #365, .T. ) ;
#6626=ORIENTED_EDGE ( 'NONE', *, *, #5905, .F. ) ;
#6629=DIRECTION ( 'NONE',  ( 0.000000000000000000, 1.000000000000000000, 0.000000000000000000 ) ) ;
#6665=VERTEX_POINT ( 'NONE', #8404 ) ;
#6675=CARTESIAN_POINT ( 'NONE',  ( 0.000000000000000000, 265.0000000000000000, 0.000000000000000000 ) ) ;
#6701=ORIENTED_EDGE ( 'NONE', *, *, #7862, .T. ) ;
#6724=EDGE_CURVE ( 'NONE', #9423, #10953, #5676, .T. ) ;
#6727=DIRECTION ( 'NONE',  ( 0.000000000000000000, 1.000000000000000000, 0.000000000000000000 ) ) ;
#6738=CIRCLE ( 'NONE', #4146, 5.000000000000004441 ) ;
#6767=ORIENTED_EDGE ( 'NONE', *, *, #3540, .F. ) ;
#6774=CARTESIAN_POINT ( 'NONE',  ( 1.377727649040772626E-14, 345.0000000000000568, -110.0000000000000284 ) ) ;
#6805=VECTOR ( 'NONE', #1475, 1000.000000000000000 ) ;
#6813=EDGE_LOOP ( 'NONE', ( #9550, #6767 ) ) ;
#6822=ORIENTED_EDGE ( 'NONE', *, *, #559, .T. ) ;
#6843=VERTEX_POINT ( 'NONE', #9584 ) ;
#6867=ORIENTED_EDGE ( 'NONE', *, *, #1080, .T. ) ;
#6870=CIRCLE ( 'NONE', #5682, 110.0000000000000284 ) ;
#6895=CARTESIAN_POINT ( 'NONE',  ( -25.00000000000000000, 345.0000000000000568, -24.99999999999998934 ) ) ;
#6914=CYLINDRICAL_SURFACE ( 'NONE', #10314, 30.00000000000000711 ) ;
#6918=CARTESIAN_POINT ( 'NONE',  ( 0.000000000000000000, 290.0000000000000568, 0.000000000000000000 ) ) ;
#6958=DIRECTION ( 'NONE',  ( 0.000000000000000000, 1.000000000000000000, 0.000000000000000000 ) ) ;
#6961=( NAMED_UNIT ( * ) SI_UNIT ( $, .STERADIAN. ) SOLID_ANGLE_UNIT ( ) );
#6975=LINE ( 'NONE', #9645, #4498 ) ;
#6976=EDGE_LOOP ( 'NONE', ( #4689, #6225, #8701, #5169 ) ) ;
#7000=CIRCLE ( 'NONE', #8581, 30.00000000000000355 ) ;
#7008=CARTESIAN_POINT ( 'NONE',  ( 1.347111479062088996E-14, 340.0000000000000000, 110.0000000000000284 ) ) ;
#7029=ORIENTED_EDGE ( 'NONE', *, *, #10585, .F. ) ;
#7033=DIRECTION ( 'NONE',  ( 1.224646799147349509E-16, 0.000000000000000000, -1.000000000000000000 ) ) ;
#7046=EDGE_LOOP ( 'NONE', ( #6524, #1196, #10982, #2959 ) ) ;
#7051=DIRECTION ( 'NONE',  ( -1.000000000000000000, 0.000000000000000000, 0.000000000000000000 ) ) ;
#7062=AXIS2_PLACEMENT_3D ( 'NONE', #1488, #1427, #10834 ) ;
#7063=VECTOR ( 'NONE', #2476, 1000.000000000000000 ) ;
#7093=CIRCLE ( 'NONE', #112, 25.00000000000000000 ) ;
#7103=AXIS2_PLACEMENT_3D ( 'NONE', #11500, #962, #3758 ) ;
#7105=VERTEX_POINT ( 'NONE', #7286 ) ;
#7107=EDGE_CURVE ( 'NONE', #3955, #4409, #10263, .T. ) ;
#7117=CARTESIAN_POINT ( 'NONE',  ( 25.00000000000000000, 445.0000000000000568, -29.99999999999998934 ) ) ;
#7135=CIRCLE ( 'NONE', #9110, 105.0000000000000284 ) ;
#7139=UNCERTAINTY_MEASURE_WITH_UNIT (LENGTH_MEASURE( 1.000000000000000082E-05 ), #2285, 'distance_accuracy_value', 'NONE');
#7152=CARTESIAN_POINT ( 'NONE',  ( 25.00000000000000000, 445.0000000000000568, -29.99999999999998934 ) ) ;
#7160=VERTEX_POINT ( 'NONE', #8202 ) ;
#7161=CIRCLE ( 'NONE', #799, 115.0000000000000284 ) ;
#7177=CIRCLE ( 'NONE', #1610, 110.0000000000000284 ) ;
#7233=VERTEX_POINT ( 'NONE', #6774 ) ;
#7256=AXIS2_PLACEMENT_3D ( 'NONE', #414, #8009, #3286 ) ;
#7285=ORIENTED_EDGE ( 'NONE', *, *, #6054, .F. ) ;
#7286=CARTESIAN_POINT ( 'NONE',  ( 1.224646799147353533E-14, 265.0000000000000000, -100.0000000000000284 ) ) ;
#7345=CYLINDRICAL_SURFACE ( 'NONE', #10375, 115.0000000000000284 ) ;
#7382=DIRECTION ( 'NONE',  ( -0.000000000000000000, -1.000000000000000000, -0.000000000000000000 ) ) ;
#7416=DIRECTION ( 'NONE',  ( 0.000000000000000000, 1.000000000000000000, 0.000000000000000000 ) ) ;
#7431=CARTESIAN_POINT ( 'NONE',  ( 0.000000000000000000, 265.0000000000000000, 0.000000000000000000 ) ) ;
#7441=ORIENTED_EDGE ( 'NONE', *, *, #4266, .T. ) ;
#7450=VERTEX_POINT ( 'NONE', #8004 ) ;
#7464=DIRECTION ( 'NONE',  ( -0.000000000000000000, -1.000000000000000000, -0.000000000000000000 ) ) ;
#7506=CARTESIAN_POINT ( 'NONE',  ( 0.000000000000000000, 345.0000000000000568, 0.000000000000000000 ) ) ;
#7544=EDGE_LOOP ( 'NONE', ( #8817, #971 ) ) ;
#7565=DIRECTION ( 'NONE',  ( -1.000000000000000000, 0.000000000000000000, -0.000000000000000000 ) ) ;
#7584=CIRCLE ( 'NONE', #2213, 115.0000000000000284 ) ;
#7591=ADVANCED_FACE ( 'NONE', ( #11198 ), #3468, .T. ) ;
#7593=AXIS2_PLACEMENT_3D ( 'NONE', #3313, #3442, #3497 ) ;
#7622=EDGE_LOOP ( 'NONE', ( #11192, #9797 ) ) ;
#7638=FACE_OUTER_BOUND ( 'NONE', #3080, .T. ) ;
#7643=APPLICATION_CONTEXT ( 'automotive_design' ) ;
#7664=ORIENTED_EDGE ( 'NONE', *, *, #3001, .T. ) ;
#7669=DIRECTION ( 'NONE',  ( 0.000000000000000000, 0.000000000000000000, 1.000000000000000000 ) ) ;
#7694=DIRECTION ( 'NONE',  ( -0.000000000000000000, 1.000000000000000000, -0.000000000000000000 ) ) ;
#7707=EDGE_LOOP ( 'NONE', ( #1193, #1317 ) ) ;
#7722=CARTESIAN_POINT ( 'NONE',  ( 1.285879139104721107E-14, 335.0000000000000000, -105.0000000000000284 ) ) ;
#7756=DIRECTION ( 'NONE',  ( 1.000000000000000000, 0.000000000000000000, 0.000000000000000000 ) ) ;
#7780=PRODUCT_DEFINITION ( 'UNKNOWN', '', #7924, #6014 ) ;
#7823=DIRECTION ( 'NONE',  ( 0.000000000000000000, 0.000000000000000000, 1.000000000000000000 ) ) ;
#7824=ORIENTED_EDGE ( 'NONE', *, *, #11486, .T. ) ;
#7830=ORIENTED_EDGE ( 'NONE', *, *, #10765, .F. ) ;
#7846=CARTESIAN_POINT ( 'NONE',  ( 0.000000000000000000, 285.0000000000000568, 0.000000000000000000 ) ) ;
#7847=FACE_OUTER_BOUND ( 'NONE', #4451, .T. ) ;
#7862=EDGE_CURVE ( 'NONE', #10543, #4650, #4634, .T. ) ;
#7869=AXIS2_PLACEMENT_3D ( 'NONE', #8512, #2916, #1977 ) ;
#7900=DIRECTION ( 'NONE',  ( 0.000000000000000000, 0.000000000000000000, 1.000000000000000000 ) ) ;
#7901=ORIENTED_EDGE ( 'NONE', *, *, #5402, .T. ) ;
#7918=LINE ( 'NONE', #7117, #2858 ) ;
#7924=PRODUCT_DEFINITION_FORMATION_WITH_SPECIFIED_SOURCE ( 'ANY', '', #1899, .NOT_KNOWN. ) ;
#7941=CARTESIAN_POINT ( 'NONE',  ( 25.00000000000000000, 445.0000000000000568, -59.99999999999999289 ) ) ;
#7945=FILL_AREA_STYLE ('',( #11706 ) ) ;
#7952=VECTOR ( 'NONE', #7565, 1000.000000000000000 ) ;
#7953=ADVANCED_FACE ( 'NONE', ( #10473 ), #9389, .F. ) ;
#7966=ORIENTED_EDGE ( 'NONE', *, *, #10617, .F. ) ;
#7975=CIRCLE ( 'NONE', #5805, 105.0000000000000284 ) ;
#8004=CARTESIAN_POINT ( 'NONE',  ( 0.000000000000000000, 335.0000000000000000, -110.0000000000000284 ) ) ;
#8009=DIRECTION ( 'NONE',  ( 0.000000000000000000, 0.000000000000000000, -1.000000000000000000 ) ) ;
#8021=FACE_OUTER_BOUND ( 'NONE', #7707, .T. ) ;
#8042=VERTEX_POINT ( 'NONE', #1648 ) ;
#8048=EDGE_LOOP ( 'NONE', ( #839, #8946, #8694, #1495 ) ) ;
#8056=DIRECTION ( 'NONE',  ( 0.000000000000000000, -0.000000000000000000, 1.000000000000000000 ) ) ;
#8059=COLOUR_RGB ( '', 0.08235294, 0.09019608, 0.10196078) ;
#8065=EDGE_CURVE ( 'NONE', #8042, #3955, #1315, .T. ) ;
#8081=ORIENTED_EDGE ( 'NONE', *, *, #9975, .T. ) ;
#8098=CARTESIAN_POINT ( 'NONE',  ( 24.99999999999999645, 345.0000000000000568, -95.00000000000000000 ) ) ;
#8117=EDGE_CURVE ( 'NONE', #7450, #1669, #9467, .T. ) ;
#8123=ORIENTED_EDGE ( 'NONE', *, *, #4213, .F. ) ;
#8125=LINE ( 'NONE', #11947, #8227 ) ;
#8148=DIRECTION ( 'NONE',  ( -0.000000000000000000, -1.000000000000000000, -0.000000000000000000 ) ) ;
#8156=ORIENTED_EDGE ( 'NONE', *, *, #3981, .T. ) ;
#8169=EDGE_CURVE ( 'NONE', #12281, #9396, #6975, .T. ) ;
#8171=EDGE_CURVE ( 'NONE', #4650, #10543, #2514, .T. ) ;
#8188=AXIS2_PLACEMENT_3D ( 'NONE', #795, #3906, #8439 ) ;
#8195=CARTESIAN_POINT ( 'NONE',  ( -25.00000000000000000, 345.0000000000000568, -29.99999999999999289 ) ) ;
#8202=CARTESIAN_POINT ( 'NONE',  ( 1.316495309083405051E-14, 340.0000000000000000, -105.0000000000000284 ) ) ;
#8217=LINE ( 'NONE', #11035, #868 ) ;
#8224=CARTESIAN_POINT ( 'NONE',  ( -25.00000000000000000, 445.0000000000000568, -29.99999999999999289 ) ) ;
#8227=VECTOR ( 'NONE', #7694, 1000.000000000000000 ) ;
#8264=DIRECTION ( 'NONE',  ( 0.000000000000000000, 1.000000000000000000, 0.000000000000000000 ) ) ;
#8267=EDGE_LOOP ( 'NONE', ( #10161, #3684, #6623, #10654 ) ) ;
#8288=DIRECTION ( 'NONE',  ( 0.000000000000000000, 0.000000000000000000, -1.000000000000000000 ) ) ;
#8305=DIRECTION ( 'NONE',  ( 0.000000000000000000, 1.000000000000000000, 0.000000000000000000 ) ) ;
#8311=FILL_AREA_STYLE_COLOUR ( '', #11744 ) ;
#8316=CARTESIAN_POINT ( 'NONE',  ( 0.000000000000000000, 285.0000000000000568, 100.0000000000000284 ) ) ;
#8360=CARTESIAN_POINT ( 'NONE',  ( 1.408343819019456413E-14, 290.0000000000000568, 115.0000000000000284 ) ) ;
#8396=CARTESIAN_POINT ( 'NONE',  ( 0.000000000000000000, 340.0000000000000000, 0.000000000000000000 ) ) ;
#8404=CARTESIAN_POINT ( 'NONE',  ( 0.000000000000000000, 340.0000000000000000, -115.0000000000000284 ) ) ;
#8408=ORIENTED_EDGE ( 'NONE', *, *, #11109, .F. ) ;
#8439=DIRECTION ( 'NONE',  ( 1.000000000000000000, 0.000000000000000000, 0.000000000000000000 ) ) ;
#8443=FACE_OUTER_BOUND ( 'NONE', #2643, .T. ) ;
#8478=CARTESIAN_POINT ( 'NONE',  ( 0.000000000000000000, 340.0000000000000000, 0.000000000000000000 ) ) ;
#8480=EDGE_LOOP ( 'NONE', ( #7830, #7664, #6701, #4968 ) ) ;
#8512=CARTESIAN_POINT ( 'NONE',  ( 0.000000000000000000, 345.0000000000000568, 0.000000000000000000 ) ) ;
#8522=CARTESIAN_POINT ( 'NONE',  ( -25.00000000000000000, 345.0000000000000568, -24.99999999999998934 ) ) ;
#8528=CARTESIAN_POINT ( 'NONE',  ( -25.00000000000000000, 345.0000000000000568, -59.99999999999999289 ) ) ;
#8534=AXIS2_PLACEMENT_3D ( 'NONE', #7941, #6958, #1227 ) ;
#8556=AXIS2_PLACEMENT_3D ( 'NONE', #3476, #7464, #857 ) ;
#8581=AXIS2_PLACEMENT_3D ( 'NONE', #6402, #6217, #1478 ) ;
#8594=CARTESIAN_POINT ( 'NONE',  ( 0.000000000000000000, 265.0000000000000000, 100.0000000000000284 ) ) ;
#8614=DIRECTION ( 'NONE',  ( -0.000000000000000000, -1.000000000000000000, -0.000000000000000000 ) ) ;
#8639=CARTESIAN_POINT ( 'NONE',  ( 1.224646799147353533E-14, 285.0000000000000568, -100.0000000000000284 ) ) ;
#8641=CARTESIAN_POINT ( 'NONE',  ( -25.00000000000000000, 445.0000000000000568, -59.99999999999999289 ) ) ;
#8676=LINE ( 'NONE', #4824, #9549 ) ;
#8694=ORIENTED_EDGE ( 'NONE', *, *, #3864, .T. ) ;
#8701=ORIENTED_EDGE ( 'NONE', *, *, #9975, .F. ) ;
#8712=VERTEX_POINT ( 'NONE', #6895 ) ;
#8716=PRODUCT_CONTEXT ( 'NONE', #7643, 'mechanical' ) ;
#8742=DIRECTION ( 'NONE',  ( -0.000000000000000000, -1.000000000000000000, -0.000000000000000000 ) ) ;
#8757=SURFACE_SIDE_STYLE ('',( #5103 ) ) ;
#8765=ORIENTED_EDGE ( 'NONE', *, *, #1588, .T. ) ;
#8772=DIRECTION ( 'NONE',  ( -0.000000000000000000, 1.000000000000000000, -0.000000000000000000 ) ) ;
#8817=ORIENTED_EDGE ( 'NONE', *, *, #4266, .F. ) ;
#8844=CARTESIAN_POINT ( 'NONE',  ( -25.00000000000000000, 345.0000000000000568, -90.00000000000000000 ) ) ;
#8850=CYLINDRICAL_SURFACE ( 'NONE', #10460, 35.00000000000000711 ) ;
#8940=DIRECTION ( 'NONE',  ( -0.000000000000000000, -1.000000000000000000, -0.000000000000000000 ) ) ;
#8946=ORIENTED_EDGE ( 'NONE', *, *, #11700, .F. ) ;
#8969=AXIS2_PLACEMENT_3D ( 'NONE', #1066, #11666, #3118 ) ;
#8980=VERTEX_POINT ( 'NONE', #11314 ) ;
#9049=DIRECTION ( 'NONE',  ( 0.000000000000000000, 1.000000000000000000, 0.000000000000000000 ) ) ;
#9070=EDGE_LOOP ( 'NONE', ( #6115, #7966, #10518, #6610 ) ) ;
#9088=DIRECTION ( 'NONE',  ( 0.000000000000000000, 0.000000000000000000, 1.000000000000000000 ) ) ;
#9110=AXIS2_PLACEMENT_3D ( 'NONE', #1410, #10002, #3407 ) ;
#9120=EDGE_CURVE ( 'NONE', #7233, #11110, #5721, .T. ) ;
#9146=ORIENTED_EDGE ( 'NONE', *, *, #6256, .T. ) ;
#9190=FACE_OUTER_BOUND ( 'NONE', #3898, .T. ) ;
#9217=DIRECTION ( 'NONE',  ( 0.000000000000000000, 0.000000000000000000, 1.000000000000000000 ) ) ;
#9232=ORIENTED_EDGE ( 'NONE', *, *, #5402, .F. ) ;
#9255=CYLINDRICAL_SURFACE ( 'NONE', #11158, 115.0000000000000284 ) ;
#9256=CIRCLE ( 'NONE', #1911, 115.0000000000000284 ) ;
#9286=ORIENTED_EDGE ( 'NONE', *, *, #2595, .F. ) ;
#9299=DIRECTION ( 'NONE',  ( 0.000000000000000000, 1.000000000000000000, 0.000000000000000000 ) ) ;
#9306=CYLINDRICAL_SURFACE ( 'NONE', #2262, 95.00000000000002842 ) ;
#9324=FACE_OUTER_BOUND ( 'NONE', #11379, .T. ) ;
#9328=CARTESIAN_POINT ( 'NONE',  ( -25.00000000000000000, 345.0000000000000568, -29.99999999999999289 ) ) ;
#9355=VECTOR ( 'NONE', #5109, 1000.000000000000000 ) ;
#9363=SHAPE_REPRESENTATION_RELATIONSHIP ( 'NONE' , 'NONE' ,  #10952, #11228 ) ;
#9375=FACE_OUTER_BOUND ( 'NONE', #6357, .T. ) ;
#9387=ADVANCED_FACE ( 'NONE', ( #569 ), #9886, .T. ) ;
#9389=TOROIDAL_SURFACE ( 'NONE', #4030, 105.0000000000000284, 5.000000000000000000 ) ;
#9396=VERTEX_POINT ( 'NONE', #11170 ) ;
#9423=VERTEX_POINT ( 'NONE', #11234 ) ;
#9424=VECTOR ( 'NONE', #8742, 1000.000000000000000 ) ;
#9447=VERTEX_POINT ( 'NONE', #3563 ) ;
#9467=CIRCLE ( 'NONE', #11677, 110.0000000000000284 ) ;
#9495=CYLINDRICAL_SURFACE ( 'NONE', #1238, 25.00000000000000000 ) ;
#9519=ORIENTED_EDGE ( 'NONE', *, *, #6256, .F. ) ;
#9549=VECTOR ( 'NONE', #8614, 1000.000000000000000 ) ;
#9550=ORIENTED_EDGE ( 'NONE', *, *, #1516, .F. ) ;
#9554=FACE_OUTER_BOUND ( 'NONE', #768, .T. ) ;
#9558=CARTESIAN_POINT ( 'NONE',  ( 0.000000000000000000, 340.0000000000000000, 105.0000000000000284 ) ) ;
#9562=CARTESIAN_POINT ( 'NONE',  ( 0.000000000000000000, 0.000000000000000000, 0.000000000000000000 ) ) ;
#9583=LINE ( 'NONE', #11347, #11320 ) ;
#9584=CARTESIAN_POINT ( 'NONE',  ( 1.347111479062088996E-14, 290.0000000000000568, 110.0000000000000284 ) ) ;
#9620=ADVANCED_FACE ( 'NONE', ( #11209 ), #7345, .T. ) ;
#9629=DIRECTION ( 'NONE',  ( -0.000000000000000000, 1.000000000000000000, -0.000000000000000000 ) ) ;
#9631=LINE ( 'NONE', #1110, #93 ) ;
#9645=CARTESIAN_POINT ( 'NONE',  ( -25.00000000000000000, 445.0000000000000568, -95.00000000000000000 ) ) ;
#9649=( GEOMETRIC_REPRESENTATION_CONTEXT ( 3 ) GLOBAL_UNCERTAINTY_ASSIGNED_CONTEXT ( ( #7139 ) ) GLOBAL_UNIT_ASSIGNED_CONTEXT ( ( #2285, #3097, #6961 ) ) REPRESENTATION_CONTEXT ( 'NONE', 'WORKASPACE' ) );
#9666=FACE_OUTER_BOUND ( 'NONE', #6250, .T. ) ;
#9765=AXIS2_PLACEMENT_3D ( 'NONE', #6675, #5927, #1940 ) ;
#9774=CYLINDRICAL_SURFACE ( 'NONE', #5264, 30.00000000000000711 ) ;
#9797=ORIENTED_EDGE ( 'NONE', *, *, #10765, .T. ) ;
#9839=EDGE_CURVE ( 'NONE', #6431, #11751, #7000, .T. ) ;
#9886=TOROIDAL_SURFACE ( 'NONE', #3528, 110.0000000000000284, 5.000000000000000000 ) ;
#9897=ADVANCED_FACE ( 'NONE', ( #4586, #9375 ), #5534, .F. ) ;
#9900=ORIENTED_EDGE ( 'NONE', *, *, #1958, .F. ) ;
#9915=ADVANCED_FACE ( 'NONE', ( #7638 ), #12323, .T. ) ;
#9944=ADVANCED_FACE ( 'NONE', ( #2904 ), #9495, .F. ) ;
#9946=APPLICATION_CONTEXT ( 'automotive_design' ) ;
#9975=EDGE_CURVE ( 'NONE', #1004, #6843, #7177, .T. ) ;
#9990=VERTEX_POINT ( 'NONE', #10564 ) ;
#10002=DIRECTION ( 'NONE',  ( -0.000000000000000000, -1.000000000000000000, -0.000000000000000000 ) ) ;
#10017=ORIENTED_EDGE ( 'NONE', *, *, #749, .F. ) ;
#10027=ORIENTED_EDGE ( 'NONE', *, *, #4115, .F. ) ;
#10033=DIRECTION ( 'NONE',  ( 0.000000000000000000, 1.000000000000000000, 0.000000000000000000 ) ) ;
#10038=CARTESIAN_POINT ( 'NONE',  ( 1.163414459189985959E-14, 290.0000000000000568, -95.00000000000002842 ) ) ;
#10087=ORIENTED_EDGE ( 'NONE', *, *, #3001, .F. ) ;
#10107=VERTEX_POINT ( 'NONE', #5091 ) ;
#10128=CIRCLE ( 'NONE', #8534, 30.00000000000000355 ) ;
#10140=DIRECTION ( 'NONE',  ( 0.000000000000000000, 1.000000000000000000, 0.000000000000000000 ) ) ;
#10142=CARTESIAN_POINT ( 'NONE',  ( 1.163414459189985959E-14, 265.0000000000000000, -95.00000000000002842 ) ) ;
#10157=AXIS2_PLACEMENT_3D ( 'NONE', #7506, #6629, #1713 ) ;
#10161=ORIENTED_EDGE ( 'NONE', *, *, #3655, .F. ) ;
#10164=VECTOR ( 'NONE', #10657, 1000.000000000000000 ) ;
#10180=ADVANCED_FACE ( 'NONE', ( #6567, #2826 ), #12129, .T. ) ;
#10200=CARTESIAN_POINT ( 'NONE',  ( -25.00000000000000000, 345.0000000000000568, -95.00000000000000000 ) ) ;
#10204=CYLINDRICAL_SURFACE ( 'NONE', #3874, 100.0000000000000284 ) ;
#10263=LINE ( 'NONE', #5542, #11631 ) ;
#10270=EDGE_LOOP ( 'NONE', ( #3555, #11594, #5255, #12249 ) ) ;
#10275=ORIENTED_EDGE ( 'NONE', *, *, #5181, .F. ) ;
#10310=CARTESIAN_POINT ( 'NONE',  ( 0.000000000000000000, 265.0000000000000000, 0.000000000000000000 ) ) ;
#10314=AXIS2_PLACEMENT_3D ( 'NONE', #4393, #4984, #12078 ) ;
#10315=DIRECTION ( 'NONE',  ( 0.000000000000000000, 1.000000000000000000, 0.000000000000000000 ) ) ;
#10356=ORIENTED_EDGE ( 'NONE', *, *, #1751, .F. ) ;
#10360=ORIENTED_EDGE ( 'NONE', *, *, #11584, .T. ) ;
#10375=AXIS2_PLACEMENT_3D ( 'NONE', #11143, #2601, #1668 ) ;
#10383=UNCERTAINTY_MEASURE_WITH_UNIT (LENGTH_MEASURE( 1.000000000000000082E-05 ), #463, 'distance_accuracy_value', 'NONE');
#10392=CARTESIAN_POINT ( 'NONE',  ( 0.000000000000000000, 340.0000000000000000, -59.99999999999999289 ) ) ;
#10402=CARTESIAN_POINT ( 'NONE',  ( 1.224646799147353533E-14, 265.0000000000000000, -100.0000000000000284 ) ) ;
#10427=ADVANCED_FACE ( 'NONE', ( #72, #6004 ), #2951, .F. ) ;
#10460=AXIS2_PLACEMENT_3D ( 'NONE', #319, #1020, #10547 ) ;
#10473=FACE_OUTER_BOUND ( 'NONE', #11965, .T. ) ;
#10518=ORIENTED_EDGE ( 'NONE', *, *, #91, .F. ) ;
#10522=DIRECTION ( 'NONE',  ( -0.000000000000000000, -1.000000000000000000, -0.000000000000000000 ) ) ;
#10532=DIRECTION ( 'NONE',  ( 0.000000000000000000, 0.000000000000000000, 1.000000000000000000 ) ) ;
#10543=VERTEX_POINT ( 'NONE', #10038 ) ;
#10547=DIRECTION ( 'NONE',  ( 0.000000000000000000, 0.000000000000000000, -1.000000000000000000 ) ) ;
#10558=LINE ( 'NONE', #910, #3465 ) ;
#10564=CARTESIAN_POINT ( 'NONE',  ( 0.000000000000000000, 285.0000000000000568, -115.0000000000000284 ) ) ;
#10585=EDGE_CURVE ( 'NONE', #2064, #7160, #7975, .T. ) ;
#10596=DIRECTION ( 'NONE',  ( 1.000000000000000000, 0.000000000000000000, 0.000000000000000000 ) ) ;
#10617=EDGE_CURVE ( 'NONE', #343, #8712, #766, .T. ) ;
#10653=DIRECTION ( 'NONE',  ( -1.000000000000000000, 0.000000000000000000, 0.000000000000000000 ) ) ;
#10654=ORIENTED_EDGE ( 'NONE', *, *, #1516, .T. ) ;
#10655=STYLED_ITEM ( 'NONE', ( #2342 ), #4709 ) ;
#10657=DIRECTION ( 'NONE',  ( 0.000000000000000000, 1.000000000000000000, 0.000000000000000000 ) ) ;
#10684=CARTESIAN_POINT ( 'NONE',  ( 0.000000000000000000, 285.0000000000000568, 0.000000000000000000 ) ) ;
#10691=ORIENTED_EDGE ( 'NONE', *, *, #10829, .F. ) ;
#10716=CARTESIAN_POINT ( 'NONE',  ( 0.000000000000000000, 285.0000000000000568, 0.000000000000000000 ) ) ;
#10734=ORIENTED_EDGE ( 'NONE', *, *, #3004, .F. ) ;
#10748=CIRCLE ( 'NONE', #5379, 30.00000000000000355 ) ;
#10765=EDGE_CURVE ( 'NONE', #11680, #9447, #11377, .T. ) ;
#10769=CARTESIAN_POINT ( 'NONE',  ( 0.000000000000000000, 265.0000000000000000, 95.00000000000002842 ) ) ;
#10771=AXIS2_PLACEMENT_3D ( 'NONE', #10716, #2869, #7669 ) ;
#10797=EDGE_CURVE ( 'NONE', #7105, #6133, #623, .T. ) ;
#10802=ORIENTED_EDGE ( 'NONE', *, *, #6054, .T. ) ;
#10829=EDGE_CURVE ( 'NONE', #6133, #4828, #4114, .T. ) ;
#10831=EDGE_CURVE ( 'NONE', #2607, #6665, #7584, .T. ) ;
#10834=DIRECTION ( 'NONE',  ( 0.000000000000000000, 0.000000000000000000, 1.000000000000000000 ) ) ;
#10853=CARTESIAN_POINT ( 'NONE',  ( 0.000000000000000000, 265.0000000000000000, 0.000000000000000000 ) ) ;
#10865=CARTESIAN_POINT ( 'NONE',  ( 0.000000000000000000, 290.0000000000000568, -110.0000000000000284 ) ) ;
#10868=EDGE_CURVE ( 'NONE', #11220, #4828, #11782, .T. ) ;
#10873=ADVANCED_FACE ( 'NONE', ( #7847 ), #2024, .T. ) ;
#10885=DIRECTION ( 'NONE',  ( 0.000000000000000000, -0.000000000000000000, 1.000000000000000000 ) ) ;
#10897=FACE_BOUND ( 'NONE', #5157, .T. ) ;
#10902=ORIENTED_EDGE ( 'NONE', *, *, #338, .F. ) ;
#10914=DIRECTION ( 'NONE',  ( -0.000000000000000000, -1.000000000000000000, -0.000000000000000000 ) ) ;
#10930=FACE_BOUND ( 'NONE', #173, .T. ) ;
#10938=AXIS2_PLACEMENT_3D ( 'NONE', #5670, #10140, #1618 ) ;
#10946=PLANE ( 'NONE',  #7256 ) ;
#10952=SHAPE_REPRESENTATION ( 'Locking Bowl Cover with Feed Chute', ( #1612 ), #3176 ) ;
#10953=VERTEX_POINT ( 'NONE', #11852 ) ;
#10969=CIRCLE ( 'NONE', #7593, 115.0000000000000284 ) ;
#10982=ORIENTED_EDGE ( 'NONE', *, *, #3540, .T. ) ;
#11020=ORIENTED_EDGE ( 'NONE', *, *, #11812, .F. ) ;
#11028=ORIENTED_EDGE ( 'NONE', *, *, #10797, .F. ) ;
#11035=CARTESIAN_POINT ( 'NONE',  ( 0.000000000000000000, 340.0000000000000000, -110.0000000000000284 ) ) ;
#11069=SURFACE_STYLE_FILL_AREA ( #6452 ) ;
#11109=EDGE_CURVE ( 'NONE', #6665, #2607, #7161, .T. ) ;
#11110=VERTEX_POINT ( 'NONE', #12158 ) ;
#11140=DIRECTION ( 'NONE',  ( 0.000000000000000000, 0.000000000000000000, -1.000000000000000000 ) ) ;
#11143=CARTESIAN_POINT ( 'NONE',  ( 0.000000000000000000, 290.0000000000000568, 0.000000000000000000 ) ) ;
#11155=EDGE_LOOP ( 'NONE', ( #3136, #11507, #6320, #1103 ) ) ;
#11158=AXIS2_PLACEMENT_3D ( 'NONE', #4590, #920, #6342 ) ;
#11170=CARTESIAN_POINT ( 'NONE',  ( -25.00000000000000000, 445.0000000000000568, -95.00000000000000000 ) ) ;
#11192=ORIENTED_EDGE ( 'NONE', *, *, #5181, .T. ) ;
#11197=EDGE_CURVE ( 'NONE', #4302, #10953, #2770, .T. ) ;
#11198=FACE_OUTER_BOUND ( 'NONE', #3069, .T. ) ;
#11209=FACE_OUTER_BOUND ( 'NONE', #7046, .T. ) ;
#11218=DIRECTION ( 'NONE',  ( 0.000000000000000000, 0.000000000000000000, 1.000000000000000000 ) ) ;
#11220=VERTEX_POINT ( 'NONE', #8639 ) ;
#11228=ADVANCED_BREP_SHAPE_REPRESENTATION ( '', ( #4709, #1612 ), #3176 ) ;
#11234=CARTESIAN_POINT ( 'NONE',  ( 25.00000000000000000, 445.0000000000000568, -90.00000000000000000 ) ) ;
#11271=CARTESIAN_POINT ( 'NONE',  ( 0.000000000000000000, 290.0000000000000568, 0.000000000000000000 ) ) ;
#11314=CARTESIAN_POINT ( 'NONE',  ( -25.00000000000000000, 445.0000000000000568, -90.00000000000000000 ) ) ;
#11320=VECTOR ( 'NONE', #6727, 1000.000000000000000 ) ;
#11347=CARTESIAN_POINT ( 'NONE',  ( 1.163414459189985959E-14, 265.0000000000000000, -95.00000000000002842 ) ) ;
#11357=PLANE ( 'NONE',  #11836 ) ;
#11365=CARTESIAN_POINT ( 'NONE',  ( 1.408343819019456413E-14, 340.0000000000000000, 115.0000000000000284 ) ) ;
#11374=LINE ( 'NONE', #12, #7952 ) ;
#11377=CIRCLE ( 'NONE', #9765, 95.00000000000002842 ) ;
#11379=EDGE_LOOP ( 'NONE', ( #258, #450, #1381, #4730 ) ) ;
#11390=CARTESIAN_POINT ( 'NONE',  ( 0.000000000000000000, 265.0000000000000000, 0.000000000000000000 ) ) ;
#11411=ORIENTED_EDGE ( 'NONE', *, *, #5064, .T. ) ;
#11425=CARTESIAN_POINT ( 'NONE',  ( 0.000000000000000000, 340.0000000000000000, -34.99999999999999289 ) ) ;
#11432=AXIS2_PLACEMENT_3D ( 'NONE', #8528, #3933, #10596 ) ;
#11457=CIRCLE ( 'NONE', #7869, 110.0000000000000284 ) ;
#11486=EDGE_CURVE ( 'NONE', #343, #366, #2142, .T. ) ;
#11500=CARTESIAN_POINT ( 'NONE',  ( 0.000000000000000000, 345.0000000000000568, 0.000000000000000000 ) ) ;
#11507=ORIENTED_EDGE ( 'NONE', *, *, #775, .F. ) ;
#11535=DIRECTION ( 'NONE',  ( 1.000000000000000000, -0.000000000000000000, 1.224646799147353207E-16 ) ) ;
#11538=LINE ( 'NONE', #10402, #6469 ) ;
#11568=DIRECTION ( 'NONE',  ( 0.000000000000000000, 1.000000000000000000, 0.000000000000000000 ) ) ;
#11584=EDGE_CURVE ( 'NONE', #2607, #11110, #4371, .T. ) ;
#11588=CARTESIAN_POINT ( 'NONE',  ( 0.000000000000000000, 290.0000000000000568, 95.00000000000002842 ) ) ;
#11590=ORIENTED_EDGE ( 'NONE', *, *, #1588, .F. ) ;
#11594=ORIENTED_EDGE ( 'NONE', *, *, #1080, .F. ) ;
#11607=SHAPE_DEFINITION_REPRESENTATION ( #1114, #10952 ) ;
#11614=AXIS2_PLACEMENT_3D ( 'NONE', #395, #3332, #2269 ) ;
#11631=VECTOR ( 'NONE', #1850, 1000.000000000000000 ) ;
#11662=CARTESIAN_POINT ( 'NONE',  ( 1.347111479062088996E-14, 340.0000000000000000, -110.0000000000000284 ) ) ;
#11666=DIRECTION ( 'NONE',  ( 0.000000000000000000, 1.000000000000000000, 0.000000000000000000 ) ) ;
#11677=AXIS2_PLACEMENT_3D ( 'NONE', #1059, #4929, #7900 ) ;
#11680=VERTEX_POINT ( 'NONE', #10142 ) ;
#11693=DIRECTION ( 'NONE',  ( 0.000000000000000000, 1.000000000000000000, 0.000000000000000000 ) ) ;
#11694=EDGE_LOOP ( 'NONE', ( #7901, #12070 ) ) ;
#11700=EDGE_CURVE ( 'NONE', #1669, #7450, #1592, .T. ) ;
#11701=( NAMED_UNIT ( * ) SI_UNIT ( $, .STERADIAN. ) SOLID_ANGLE_UNIT ( ) );
#11706=FILL_AREA_STYLE_COLOUR ( '', #8059 ) ;
#11739=ORIENTED_EDGE ( 'NONE', *, *, #3541, .T. ) ;
#11744=COLOUR_RGB ( '', 0.08235294, 0.09019608, 0.10196078) ;
#11751=VERTEX_POINT ( 'NONE', #9328 ) ;
#11772=SURFACE_STYLE_USAGE ( .BOTH. , #8757 ) ;
#11782=CIRCLE ( 'NONE', #10771, 100.0000000000000284 ) ;
#11812=EDGE_CURVE ( 'NONE', #8980, #11984, #10748, .T. ) ;
#11836=AXIS2_PLACEMENT_3D ( 'NONE', #8224, #8288, #4430 ) ;
#11852=CARTESIAN_POINT ( 'NONE',  ( 25.00000000000000000, 345.0000000000000568, -90.00000000000000000 ) ) ;
#11862=TOROIDAL_SURFACE ( 'NONE', #2263, 105.0000000000000284, 5.000000000000000000 ) ;
#11868=DIRECTION ( 'NONE',  ( 0.000000000000000000, 0.000000000000000000, 1.000000000000000000 ) ) ;
#11897=CARTESIAN_POINT ( 'NONE',  ( -25.00000000000000000, 445.0000000000000568, -95.00000000000000000 ) ) ;
#11912=ORIENTED_EDGE ( 'NONE', *, *, #5905, .T. ) ;
#11937=CARTESIAN_POINT ( 'NONE',  ( 25.00000000000000000, 445.0000000000000568, -24.99999999999998934 ) ) ;
#11943=ORIENTED_EDGE ( 'NONE', *, *, #12131, .T. ) ;
#11947=CARTESIAN_POINT ( 'NONE',  ( 3.061616997868383043E-15, 264.9990000000000236, -84.99999999999998579 ) ) ;
#11960=ADVANCED_FACE ( 'NONE', ( #5794 ), #2985, .T. ) ;
#11965=EDGE_LOOP ( 'NONE', ( #2394, #3764, #7029, #1047 ) ) ;
#11975=CIRCLE ( 'NONE', #826, 35.00000000000000000 ) ;
#11984=VERTEX_POINT ( 'NONE', #1986 ) ;
#12007=( LENGTH_UNIT ( ) NAMED_UNIT ( * ) SI_UNIT ( .MILLI., .METRE. ) );
#12026=ORIENTED_EDGE ( 'NONE', *, *, #3541, .F. ) ;
#12060=DIRECTION ( 'NONE',  ( -0.000000000000000000, -1.000000000000000000, -0.000000000000000000 ) ) ;
#12061=LINE ( 'NONE', #8360, #3697 ) ;
#12067=AXIS2_PLACEMENT_3D ( 'NONE', #5967, #10885, #1292 ) ;
#12070=ORIENTED_EDGE ( 'NONE', *, *, #10868, .T. ) ;
#12078=DIRECTION ( 'NONE',  ( 0.000000000000000000, 0.000000000000000000, -1.000000000000000000 ) ) ;
#12107=VERTEX_POINT ( 'NONE', #7152 ) ;
#12111=DIRECTION ( 'NONE',  ( 0.000000000000000000, 1.000000000000000000, 0.000000000000000000 ) ) ;
#12121=FACE_OUTER_BOUND ( 'NONE', #1485, .T. ) ;
#12129=PLANE ( 'NONE',  #10157 ) ;
#12131=EDGE_CURVE ( 'NONE', #9447, #4650, #1297, .T. ) ;
#12158=CARTESIAN_POINT ( 'NONE',  ( 0.000000000000000000, 345.0000000000000568, 110.0000000000000284 ) ) ;
#12169=DIRECTION ( 'NONE',  ( 0.000000000000000000, 0.000000000000000000, 1.000000000000000000 ) ) ;
#12170=ORIENTED_EDGE ( 'NONE', *, *, #9839, .T. ) ;
#12199=DIRECTION ( 'NONE',  ( 0.000000000000000000, 1.000000000000000000, 0.000000000000000000 ) ) ;
#12205=DIRECTION ( 'NONE',  ( 0.000000000000000000, -0.000000000000000000, 1.000000000000000000 ) ) ;
#12208=FACE_BOUND ( 'NONE', #4484, .T. ) ;
#12222=ADVANCED_FACE ( 'NONE', ( #8443 ), #6530, .F. ) ;
#12223=ORIENTED_EDGE ( 'NONE', *, *, #338, .T. ) ;
#12229=CARTESIAN_POINT ( 'NONE',  ( 0.000000000000000000, 345.0000000000000568, -59.99999999999999289 ) ) ;
#12231=ADVANCED_FACE ( 'NONE', ( #9190, #12208 ), #3715, .T. ) ;
#12235=DIRECTION ( 'NONE',  ( -0.000000000000000000, -1.000000000000000000, -0.000000000000000000 ) ) ;
#12249=ORIENTED_EDGE ( 'NONE', *, *, #10617, .T. ) ;
#12253=DIRECTION ( 'NONE',  ( 1.000000000000000000, 0.000000000000000000, 0.000000000000000000 ) ) ;
#12257=CIRCLE ( 'NONE', #2098, 25.00000000000000000 ) ;
#12260=ADVANCED_FACE ( 'NONE', ( #4711 ), #9255, .T. ) ;
#12267=DIRECTION ( 'NONE',  ( 0.000000000000000000, -0.000000000000000000, 1.000000000000000000 ) ) ;
#12277=ORIENTED_EDGE ( 'NONE', *, *, #7107, .T. ) ;
#12281=VERTEX_POINT ( 'NONE', #3657 ) ;
#12282=DIRECTION ( 'NONE',  ( 0.000000000000000000, 1.000000000000000000, 0.000000000000000000 ) ) ;
#12323=PLANE ( 'NONE',  #8188 ) ;
#12328=ADVANCED_FACE ( 'NONE', ( #6586 ), #2718, .F. ) ;
ENDSEC;
END-ISO-10303-21;
